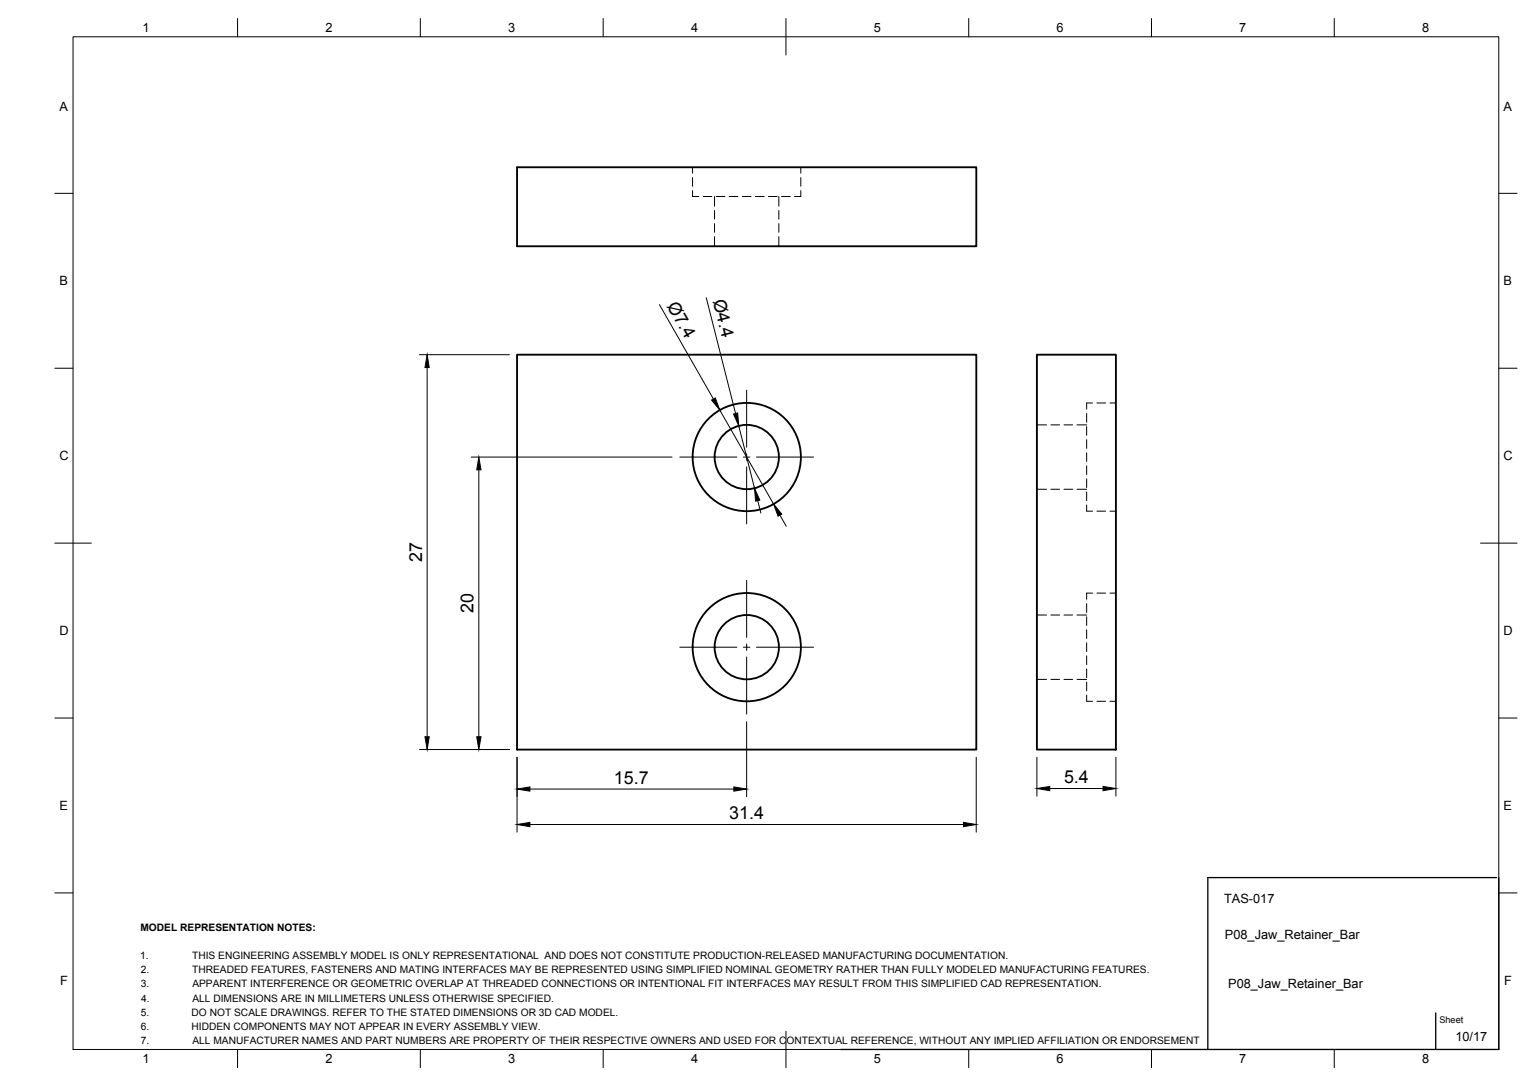
ISO-10303-21;
HEADER;
/* Generated by software containing ST-Developer
 * from STEP Tools, Inc. (www.steptools.com) 
 */

FILE_DESCRIPTION(
/* description */ ('STEP AP203'),
/* implementation_level */ '2;1');

FILE_NAME(
/* name */ 'P08_Jaw_Retainer_Bar.step',
/* time_stamp */ '2026-11-15T15:04:01-08:00',
/* author */ (''),
/* organization */ (''),
/* preprocessor_version */ 'ST-DEVELOPER v20.2',
/* originating_system */ 'Autodesk Translation Framework v15.17.0.0',
/* authorisation */ '');

FILE_SCHEMA (('AUTOMOTIVE_DESIGN { 1 0 10303 214 3 1 1 }'));
ENDSEC;

DATA;
#10=MECHANICAL_DESIGN_GEOMETRIC_PRESENTATION_REPRESENTATION('',(#288),#16598);
#210=SHAPE_REPRESENTATION_RELATIONSHIP('SRR','None',#16704,#234);
#234=ADVANCED_BREP_SHAPE_REPRESENTATION('',(#258),#16580);
#258=MANIFOLD_SOLID_BREP('Body1',#9793);
#288=STYLED_ITEM('',(#16833),#258);
#336=FACE_BOUND('',#1679,.T.);
#337=FACE_BOUND('',#1680,.T.);
#338=FACE_BOUND('',#1682,.T.);
#339=FACE_BOUND('',#1683,.T.);
#340=FACE_BOUND('',#1685,.T.);
#341=FACE_BOUND('',#1687,.T.);
#587=PLANE('',#10326);
#588=PLANE('',#10327);
#589=PLANE('',#10328);
#590=PLANE('',#10329);
#591=PLANE('',#10330);
#592=PLANE('',#10331);
#593=PLANE('',#10332);
#594=PLANE('',#10333);
#1089=FACE_OUTER_BOUND('',#1670,.T.);
#1090=FACE_OUTER_BOUND('',#1671,.T.);
#1091=FACE_OUTER_BOUND('',#1672,.T.);
#1092=FACE_OUTER_BOUND('',#1673,.T.);
#1093=FACE_OUTER_BOUND('',#1674,.T.);
#1094=FACE_OUTER_BOUND('',#1675,.T.);
#1095=FACE_OUTER_BOUND('',#1676,.T.);
#1096=FACE_OUTER_BOUND('',#1677,.T.);
#1097=FACE_OUTER_BOUND('',#1678,.T.);
#1098=FACE_OUTER_BOUND('',#1681,.T.);
#1099=FACE_OUTER_BOUND('',#1684,.T.);
#1100=FACE_OUTER_BOUND('',#1686,.T.);
#1670=EDGE_LOOP('',(#7509,#7510,#7511,#7512));
#1671=EDGE_LOOP('',(#7513,#7514,#7515,#7516));
#1672=EDGE_LOOP('',(#7517,#7518,#7519,#7520));
#1673=EDGE_LOOP('',(#7521,#7522,#7523,#7524));
#1674=EDGE_LOOP('',(#7525,#7526,#7527,#7528));
#1675=EDGE_LOOP('',(#7529,#7530,#7531,#7532));
#1676=EDGE_LOOP('',(#7533,#7534,#7535,#7536));
#1677=EDGE_LOOP('',(#7537,#7538,#7539,#7540));
#1678=EDGE_LOOP('',(#7541,#7542,#7543,#7544));
#1679=EDGE_LOOP('',(#7545));
#1680=EDGE_LOOP('',(#7546));
#1681=EDGE_LOOP('',(#7547,#7548,#7549,#7550));
#1682=EDGE_LOOP('',(#7551));
#1683=EDGE_LOOP('',(#7552));
#1684=EDGE_LOOP('',(#7553));
#1685=EDGE_LOOP('',(#7554));
#1686=EDGE_LOOP('',(#7555));
#1687=EDGE_LOOP('',(#7556));
#2540=LINE('',#14630,#3588);
#2541=LINE('',#14636,#3589);
#2542=LINE('',#14642,#3590);
#2543=LINE('',#14648,#3591);
#2544=LINE('',#14653,#3592);
#2545=LINE('',#14655,#3593);
#2546=LINE('',#14657,#3594);
#2547=LINE('',#14658,#3595);
#2548=LINE('',#14661,#3596);
#2549=LINE('',#14663,#3597);
#2550=LINE('',#14664,#3598);
#2551=LINE('',#14667,#3599);
#2552=LINE('',#14669,#3600);
#2553=LINE('',#14670,#3601);
#2554=LINE('',#14672,#3602);
#2555=LINE('',#14673,#3603);
#3588=VECTOR('',#11812,3.7);
#3589=VECTOR('',#11819,3.7);
#3590=VECTOR('',#11826,2.2);
#3591=VECTOR('',#11833,2.2);
#3592=VECTOR('',#11838,1000.);
#3593=VECTOR('',#11839,1000.);
#3594=VECTOR('',#11840,1000.);
#3595=VECTOR('',#11841,1000.);
#3596=VECTOR('',#11844,1000.);
#3597=VECTOR('',#11845,1000.);
#3598=VECTOR('',#11846,1000.);
#3599=VECTOR('',#11849,1000.);
#3600=VECTOR('',#11850,1000.);
#3601=VECTOR('',#11851,1000.);
#3602=VECTOR('',#11854,1000.);
#3603=VECTOR('',#11855,1000.);
#4275=CIRCLE('',#10315,3.7);
#4276=CIRCLE('',#10316,3.7);
#4277=CIRCLE('',#10318,3.7);
#4278=CIRCLE('',#10319,3.7);
#4279=CIRCLE('',#10321,2.2);
#4280=CIRCLE('',#10322,2.2);
#4281=CIRCLE('',#10324,2.2);
#4282=CIRCLE('',#10325,2.2);
#4759=VERTEX_POINT('',#14627);
#4760=VERTEX_POINT('',#14629);
#4761=VERTEX_POINT('',#14633);
#4762=VERTEX_POINT('',#14635);
#4763=VERTEX_POINT('',#14639);
#4764=VERTEX_POINT('',#14641);
#4765=VERTEX_POINT('',#14645);
#4766=VERTEX_POINT('',#14647);
#4767=VERTEX_POINT('',#14651);
#4768=VERTEX_POINT('',#14652);
#4769=VERTEX_POINT('',#14654);
#4770=VERTEX_POINT('',#14656);
#4771=VERTEX_POINT('',#14660);
#4772=VERTEX_POINT('',#14662);
#4773=VERTEX_POINT('',#14666);
#4774=VERTEX_POINT('',#14668);
#5767=EDGE_CURVE('',#4759,#4759,#4275,.T.);
#5768=EDGE_CURVE('',#4759,#4760,#2540,.T.);
#5769=EDGE_CURVE('',#4760,#4760,#4276,.T.);
#5770=EDGE_CURVE('',#4761,#4761,#4277,.T.);
#5771=EDGE_CURVE('',#4761,#4762,#2541,.T.);
#5772=EDGE_CURVE('',#4762,#4762,#4278,.T.);
#5773=EDGE_CURVE('',#4763,#4763,#4279,.T.);
#5774=EDGE_CURVE('',#4763,#4764,#2542,.T.);
#5775=EDGE_CURVE('',#4764,#4764,#4280,.T.);
#5776=EDGE_CURVE('',#4765,#4765,#4281,.T.);
#5777=EDGE_CURVE('',#4765,#4766,#2543,.T.);
#5778=EDGE_CURVE('',#4766,#4766,#4282,.T.);
#5779=EDGE_CURVE('',#4767,#4768,#2544,.T.);
#5780=EDGE_CURVE('',#4769,#4768,#2545,.T.);
#5781=EDGE_CURVE('',#4770,#4769,#2546,.T.);
#5782=EDGE_CURVE('',#4770,#4767,#2547,.T.);
#5783=EDGE_CURVE('',#4768,#4771,#2548,.T.);
#5784=EDGE_CURVE('',#4772,#4771,#2549,.T.);
#5785=EDGE_CURVE('',#4769,#4772,#2550,.T.);
#5786=EDGE_CURVE('',#4771,#4773,#2551,.T.);
#5787=EDGE_CURVE('',#4774,#4773,#2552,.T.);
#5788=EDGE_CURVE('',#4772,#4774,#2553,.T.);
#5789=EDGE_CURVE('',#4773,#4767,#2554,.T.);
#5790=EDGE_CURVE('',#4774,#4770,#2555,.T.);
#7509=ORIENTED_EDGE('',*,*,#5767,.T.);
#7510=ORIENTED_EDGE('',*,*,#5768,.T.);
#7511=ORIENTED_EDGE('',*,*,#5769,.F.);
#7512=ORIENTED_EDGE('',*,*,#5768,.F.);
#7513=ORIENTED_EDGE('',*,*,#5770,.T.);
#7514=ORIENTED_EDGE('',*,*,#5771,.T.);
#7515=ORIENTED_EDGE('',*,*,#5772,.F.);
#7516=ORIENTED_EDGE('',*,*,#5771,.F.);
#7517=ORIENTED_EDGE('',*,*,#5773,.T.);
#7518=ORIENTED_EDGE('',*,*,#5774,.T.);
#7519=ORIENTED_EDGE('',*,*,#5775,.F.);
#7520=ORIENTED_EDGE('',*,*,#5774,.F.);
#7521=ORIENTED_EDGE('',*,*,#5776,.T.);
#7522=ORIENTED_EDGE('',*,*,#5777,.T.);
#7523=ORIENTED_EDGE('',*,*,#5778,.F.);
#7524=ORIENTED_EDGE('',*,*,#5777,.F.);
#7525=ORIENTED_EDGE('',*,*,#5779,.T.);
#7526=ORIENTED_EDGE('',*,*,#5780,.F.);
#7527=ORIENTED_EDGE('',*,*,#5781,.F.);
#7528=ORIENTED_EDGE('',*,*,#5782,.T.);
#7529=ORIENTED_EDGE('',*,*,#5783,.T.);
#7530=ORIENTED_EDGE('',*,*,#5784,.F.);
#7531=ORIENTED_EDGE('',*,*,#5785,.F.);
#7532=ORIENTED_EDGE('',*,*,#5780,.T.);
#7533=ORIENTED_EDGE('',*,*,#5786,.T.);
#7534=ORIENTED_EDGE('',*,*,#5787,.F.);
#7535=ORIENTED_EDGE('',*,*,#5788,.F.);
#7536=ORIENTED_EDGE('',*,*,#5784,.T.);
#7537=ORIENTED_EDGE('',*,*,#5789,.T.);
#7538=ORIENTED_EDGE('',*,*,#5782,.F.);
#7539=ORIENTED_EDGE('',*,*,#5790,.F.);
#7540=ORIENTED_EDGE('',*,*,#5787,.T.);
#7541=ORIENTED_EDGE('',*,*,#5781,.T.);
#7542=ORIENTED_EDGE('',*,*,#5785,.T.);
#7543=ORIENTED_EDGE('',*,*,#5788,.T.);
#7544=ORIENTED_EDGE('',*,*,#5790,.T.);
#7545=ORIENTED_EDGE('',*,*,#5773,.F.);
#7546=ORIENTED_EDGE('',*,*,#5776,.F.);
#7547=ORIENTED_EDGE('',*,*,#5779,.F.);
#7548=ORIENTED_EDGE('',*,*,#5789,.F.);
#7549=ORIENTED_EDGE('',*,*,#5786,.F.);
#7550=ORIENTED_EDGE('',*,*,#5783,.F.);
#7551=ORIENTED_EDGE('',*,*,#5772,.T.);
#7552=ORIENTED_EDGE('',*,*,#5769,.T.);
#7553=ORIENTED_EDGE('',*,*,#5770,.F.);
#7554=ORIENTED_EDGE('',*,*,#5775,.T.);
#7555=ORIENTED_EDGE('',*,*,#5767,.F.);
#7556=ORIENTED_EDGE('',*,*,#5778,.T.);
#9189=CYLINDRICAL_SURFACE('',#10314,3.7);
#9190=CYLINDRICAL_SURFACE('',#10317,3.7);
#9191=CYLINDRICAL_SURFACE('',#10320,2.2);
#9192=CYLINDRICAL_SURFACE('',#10323,2.2);
#9414=ADVANCED_FACE('',(#1089),#9189,.F.);
#9415=ADVANCED_FACE('',(#1090),#9190,.F.);
#9416=ADVANCED_FACE('',(#1091),#9191,.F.);
#9417=ADVANCED_FACE('',(#1092),#9192,.F.);
#9418=ADVANCED_FACE('',(#1093),#587,.F.);
#9419=ADVANCED_FACE('',(#1094),#588,.F.);
#9420=ADVANCED_FACE('',(#1095),#589,.F.);
#9421=ADVANCED_FACE('',(#1096),#590,.F.);
#9422=ADVANCED_FACE('',(#1097,#336,#337),#591,.F.);
#9423=ADVANCED_FACE('',(#1098,#338,#339),#592,.T.);
#9424=ADVANCED_FACE('',(#1099,#340),#593,.F.);
#9425=ADVANCED_FACE('',(#1100,#341),#594,.F.);
#9793=CLOSED_SHELL('',(#9414,#9415,#9416,#9417,#9418,#9419,#9420,#9421,
#9422,#9423,#9424,#9425));
#10313=AXIS2_PLACEMENT_3D('',#14625,#11806,#11807);
#10314=AXIS2_PLACEMENT_3D('',#14626,#11808,#11809);
#10315=AXIS2_PLACEMENT_3D('',#14628,#11810,#11811);
#10316=AXIS2_PLACEMENT_3D('',#14631,#11813,#11814);
#10317=AXIS2_PLACEMENT_3D('',#14632,#11815,#11816);
#10318=AXIS2_PLACEMENT_3D('',#14634,#11817,#11818);
#10319=AXIS2_PLACEMENT_3D('',#14637,#11820,#11821);
#10320=AXIS2_PLACEMENT_3D('',#14638,#11822,#11823);
#10321=AXIS2_PLACEMENT_3D('',#14640,#11824,#11825);
#10322=AXIS2_PLACEMENT_3D('',#14643,#11827,#11828);
#10323=AXIS2_PLACEMENT_3D('',#14644,#11829,#11830);
#10324=AXIS2_PLACEMENT_3D('',#14646,#11831,#11832);
#10325=AXIS2_PLACEMENT_3D('',#14649,#11834,#11835);
#10326=AXIS2_PLACEMENT_3D('',#14650,#11836,#11837);
#10327=AXIS2_PLACEMENT_3D('',#14659,#11842,#11843);
#10328=AXIS2_PLACEMENT_3D('',#14665,#11847,#11848);
#10329=AXIS2_PLACEMENT_3D('',#14671,#11852,#11853);
#10330=AXIS2_PLACEMENT_3D('',#14674,#11856,#11857);
#10331=AXIS2_PLACEMENT_3D('',#14675,#11858,#11859);
#10332=AXIS2_PLACEMENT_3D('',#14676,#11860,#11861);
#10333=AXIS2_PLACEMENT_3D('',#14677,#11862,#11863);
#11806=DIRECTION('axis',(0.,0.,1.));
#11807=DIRECTION('refdir',(1.,0.,0.));
#11808=DIRECTION('center_axis',(0.,0.,-1.));
#11809=DIRECTION('ref_axis',(-1.,0.,0.));
#11810=DIRECTION('center_axis',(0.,0.,1.));
#11811=DIRECTION('ref_axis',(1.,0.,0.));
#11812=DIRECTION('',(0.,0.,-1.));
#11813=DIRECTION('center_axis',(0.,0.,1.));
#11814=DIRECTION('ref_axis',(-1.,0.,0.));
#11815=DIRECTION('center_axis',(0.,0.,-1.));
#11816=DIRECTION('ref_axis',(-1.,0.,0.));
#11817=DIRECTION('center_axis',(0.,0.,1.));
#11818=DIRECTION('ref_axis',(1.,0.,0.));
#11819=DIRECTION('',(0.,0.,-1.));
#11820=DIRECTION('center_axis',(0.,0.,1.));
#11821=DIRECTION('ref_axis',(-1.,0.,0.));
#11822=DIRECTION('center_axis',(0.,0.,-1.));
#11823=DIRECTION('ref_axis',(-1.,0.,0.));
#11824=DIRECTION('center_axis',(0.,0.,1.));
#11825=DIRECTION('ref_axis',(-1.,0.,0.));
#11826=DIRECTION('',(0.,0.,-1.));
#11827=DIRECTION('center_axis',(0.,0.,1.));
#11828=DIRECTION('ref_axis',(1.,0.,0.));
#11829=DIRECTION('center_axis',(0.,0.,-1.));
#11830=DIRECTION('ref_axis',(-1.,0.,0.));
#11831=DIRECTION('center_axis',(0.,0.,1.));
#11832=DIRECTION('ref_axis',(-1.,0.,0.));
#11833=DIRECTION('',(0.,0.,-1.));
#11834=DIRECTION('center_axis',(0.,0.,1.));
#11835=DIRECTION('ref_axis',(1.,0.,0.));
#11836=DIRECTION('center_axis',(-1.,0.,0.));
#11837=DIRECTION('ref_axis',(0.,0.,1.));
#11838=DIRECTION('',(0.,1.,0.));
#11839=DIRECTION('',(0.,0.,-1.));
#11840=DIRECTION('',(0.,1.,0.));
#11841=DIRECTION('',(0.,0.,-1.));
#11842=DIRECTION('center_axis',(0.,-1.,0.));
#11843=DIRECTION('ref_axis',(0.,0.,-1.));
#11844=DIRECTION('',(-1.,0.,0.));
#11845=DIRECTION('',(0.,0.,-1.));
#11846=DIRECTION('',(-1.,0.,0.));
#11847=DIRECTION('center_axis',(1.,0.,0.));
#11848=DIRECTION('ref_axis',(0.,0.,-1.));
#11849=DIRECTION('',(0.,-1.,0.));
#11850=DIRECTION('',(0.,0.,-1.));
#11851=DIRECTION('',(0.,-1.,0.));
#11852=DIRECTION('center_axis',(0.,1.,0.));
#11853=DIRECTION('ref_axis',(0.,0.,1.));
#11854=DIRECTION('',(1.,0.,0.));
#11855=DIRECTION('',(1.,0.,0.));
#11856=DIRECTION('center_axis',(0.,0.,-1.));
#11857=DIRECTION('ref_axis',(-1.,0.,0.));
#11858=DIRECTION('center_axis',(0.,0.,-1.));
#11859=DIRECTION('ref_axis',(-1.,0.,0.));
#11860=DIRECTION('center_axis',(0.,0.,1.));
#11861=DIRECTION('ref_axis',(1.,0.,0.));
#11862=DIRECTION('center_axis',(0.,0.,1.));
#11863=DIRECTION('ref_axis',(1.,0.,0.));
#14625=CARTESIAN_POINT('',(0.,0.,0.));
#14626=CARTESIAN_POINT('Origin',(0.,18.,74.3));
#14627=CARTESIAN_POINT('',(3.7,18.,74.3));
#14628=CARTESIAN_POINT('Origin',(0.,18.,74.3));
#14629=CARTESIAN_POINT('',(3.7,18.,72.3));
#14630=CARTESIAN_POINT('',(3.7,18.,74.3));
#14631=CARTESIAN_POINT('Origin',(0.,18.,72.3));
#14632=CARTESIAN_POINT('Origin',(0.,5.,74.3));
#14633=CARTESIAN_POINT('',(3.7,5.,74.3));
#14634=CARTESIAN_POINT('Origin',(0.,5.,74.3));
#14635=CARTESIAN_POINT('',(3.7,5.,72.3));
#14636=CARTESIAN_POINT('',(3.7,5.,74.3));
#14637=CARTESIAN_POINT('Origin',(0.,5.,72.3));
#14638=CARTESIAN_POINT('Origin',(0.,5.,78.5));
#14639=CARTESIAN_POINT('',(2.2,5.,77.7));
#14640=CARTESIAN_POINT('Origin',(0.,5.,77.7));
#14641=CARTESIAN_POINT('',(2.2,5.,74.3));
#14642=CARTESIAN_POINT('',(2.2,5.,78.5));
#14643=CARTESIAN_POINT('Origin',(0.,5.,74.3));
#14644=CARTESIAN_POINT('Origin',(0.,18.,78.5));
#14645=CARTESIAN_POINT('',(2.2,18.,77.7));
#14646=CARTESIAN_POINT('Origin',(0.,18.,77.7));
#14647=CARTESIAN_POINT('',(2.2,18.,74.3));
#14648=CARTESIAN_POINT('',(2.2,18.,78.5));
#14649=CARTESIAN_POINT('Origin',(0.,18.,74.3));
#14650=CARTESIAN_POINT('Origin',(15.7,-2.,77.7));
#14651=CARTESIAN_POINT('',(15.7,-2.,72.3));
#14652=CARTESIAN_POINT('',(15.7,25.,72.3));
#14653=CARTESIAN_POINT('',(15.7,-2.,72.3));
#14654=CARTESIAN_POINT('',(15.7,25.,77.7));
#14655=CARTESIAN_POINT('',(15.7,25.,77.7));
#14656=CARTESIAN_POINT('',(15.7,-2.,77.7));
#14657=CARTESIAN_POINT('',(15.7,-2.,77.7));
#14658=CARTESIAN_POINT('',(15.7,-2.,77.7));
#14659=CARTESIAN_POINT('Origin',(-15.7,25.,77.7));
#14660=CARTESIAN_POINT('',(-15.7,25.,72.3));
#14661=CARTESIAN_POINT('',(-15.7,25.,72.3));
#14662=CARTESIAN_POINT('',(-15.7,25.,77.7));
#14663=CARTESIAN_POINT('',(-15.7,25.,77.7));
#14664=CARTESIAN_POINT('',(-15.7,25.,77.7));
#14665=CARTESIAN_POINT('Origin',(-15.7,-2.,77.7));
#14666=CARTESIAN_POINT('',(-15.7,-2.,72.3));
#14667=CARTESIAN_POINT('',(-15.7,-2.,72.3));
#14668=CARTESIAN_POINT('',(-15.7,-2.,77.7));
#14669=CARTESIAN_POINT('',(-15.7,-2.,77.7));
#14670=CARTESIAN_POINT('',(-15.7,-2.,77.7));
#14671=CARTESIAN_POINT('Origin',(-15.7,-2.,77.7));
#14672=CARTESIAN_POINT('',(-15.7,-2.,72.3));
#14673=CARTESIAN_POINT('',(-15.7,-2.,77.7));
#14674=CARTESIAN_POINT('Origin',(0.,0.,77.7));
#14675=CARTESIAN_POINT('Origin',(0.,0.,72.3));
#14676=CARTESIAN_POINT('Origin',(0.,5.,74.3));
#14677=CARTESIAN_POINT('Origin',(0.,18.,74.3));
#16554=UNCERTAINTY_MEASURE_WITH_UNIT(LENGTH_MEASURE(0.01),#16599,
'DISTANCE_ACCURACY_VALUE',
'Maximum model space distance between geometric entities at asserted c
onnectivities');
#16572=UNCERTAINTY_MEASURE_WITH_UNIT(LENGTH_MEASURE(0.01),#16599,
'DISTANCE_ACCURACY_VALUE',
'Maximum model space distance between geometric entities at asserted c
onnectivities');
#16580=(
GEOMETRIC_REPRESENTATION_CONTEXT(3)
GLOBAL_UNCERTAINTY_ASSIGNED_CONTEXT((#16554))
GLOBAL_UNIT_ASSIGNED_CONTEXT((#16599,#16601,#16602))
REPRESENTATION_CONTEXT('','3D')
);
#16598=(
GEOMETRIC_REPRESENTATION_CONTEXT(3)
GLOBAL_UNCERTAINTY_ASSIGNED_CONTEXT((#16572))
GLOBAL_UNIT_ASSIGNED_CONTEXT((#16599,#16601,#16602))
REPRESENTATION_CONTEXT('','3D')
);
#16599=(
LENGTH_UNIT()
NAMED_UNIT(*)
SI_UNIT(.MILLI.,.METRE.)
);
#16601=(
NAMED_UNIT(*)
PLANE_ANGLE_UNIT()
SI_UNIT($,.RADIAN.)
);
#16602=(
NAMED_UNIT(*)
SI_UNIT($,.STERADIAN.)
SOLID_ANGLE_UNIT()
);
#16610=SHAPE_DEFINITION_REPRESENTATION(#16635,#16704);
#16635=PRODUCT_DEFINITION_SHAPE('',$,#16730);
#16704=SHAPE_REPRESENTATION('',(#10313),#16580);
#16722=PRODUCT_DEFINITION_CONTEXT('part definition',#16799,'design');
#16730=PRODUCT_DEFINITION('P08_Jaw_Retainer_Bar','P08_Jaw_Retainer_Bar',
#16755,#16722);
#16755=PRODUCT_DEFINITION_FORMATION('',$,#16808);
#16799=APPLICATION_CONTEXT(
'Core Data for Automotive Mechanical Design Process');
#16800=PRODUCT_CONTEXT('part definition',#16799,'mechanical');
#16808=PRODUCT('P08_Jaw_Retainer_Bar','P08_Jaw_Retainer_Bar',$,(#16800));
#16833=PRESENTATION_STYLE_ASSIGNMENT((#16842));
#16842=SURFACE_STYLE_USAGE(.BOTH.,#16851);
#16851=SURFACE_SIDE_STYLE('',(#16860));
#16860=SURFACE_STYLE_FILL_AREA(#16869);
#16869=FILL_AREA_STYLE('Blue',(#16878));
#16878=FILL_AREA_STYLE_COLOUR('Blue',#16887);
#16887=COLOUR_RGB('Blue',0.,0.4,0.8);
ENDSEC;
END-ISO-10303-21;
